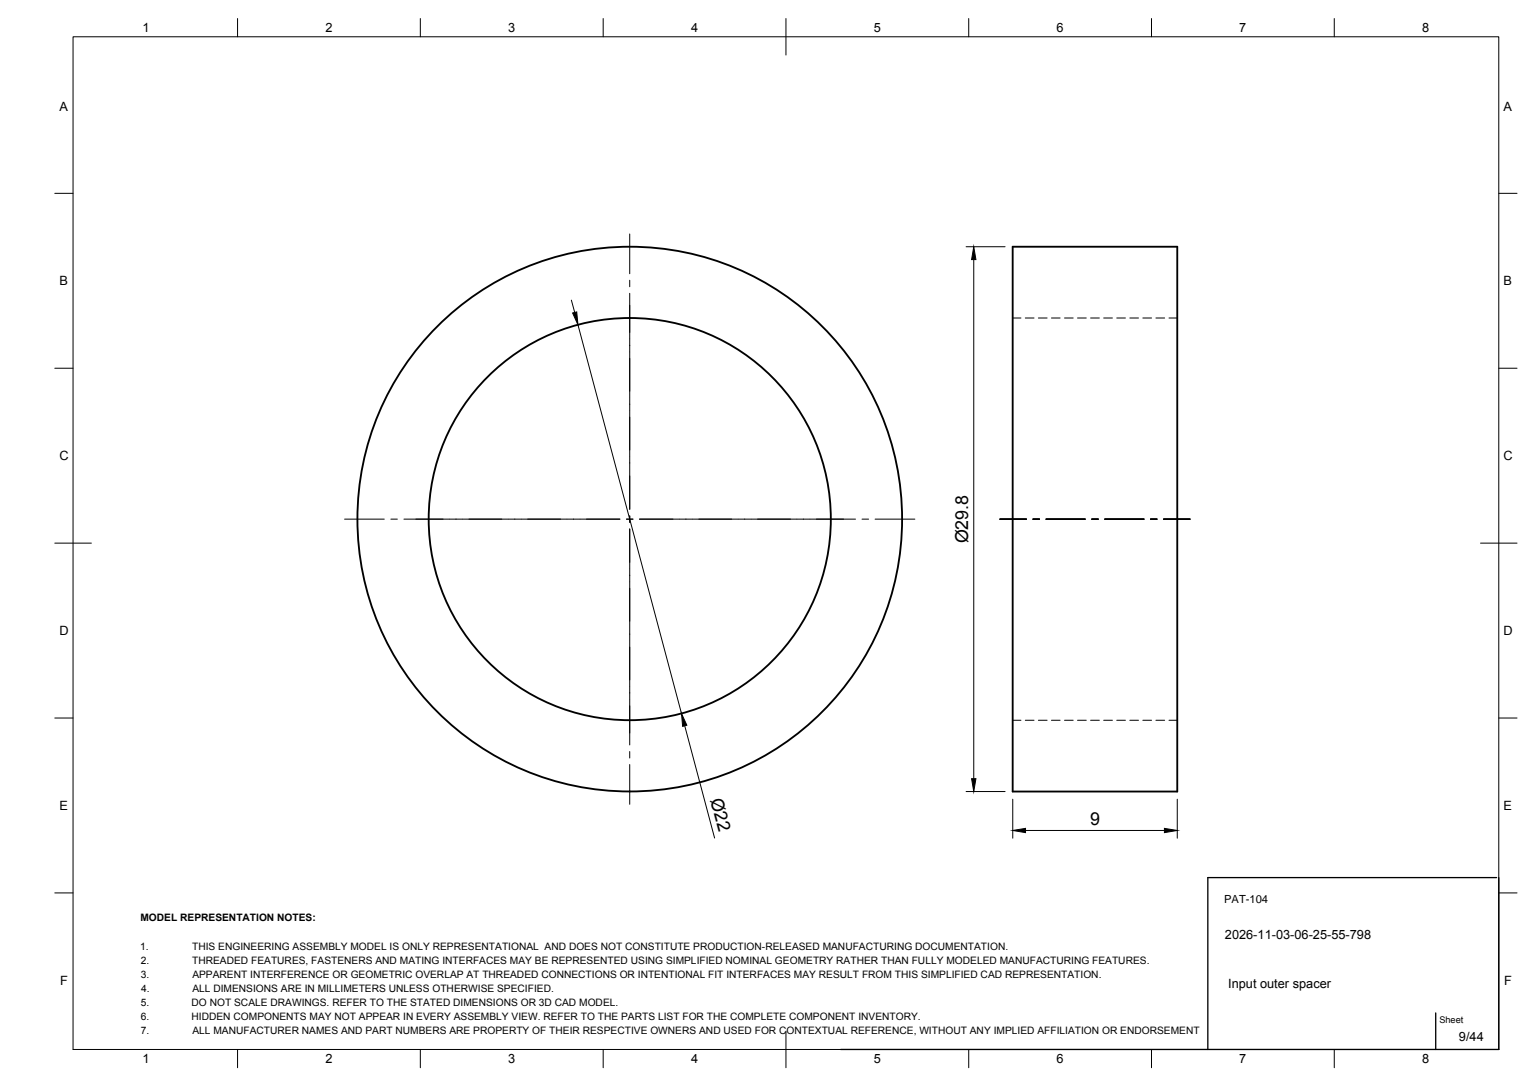
ISO-10303-21;
HEADER;
/* Generated by software containing ST-Developer
 * from STEP Tools, Inc. (www.steptools.com) 
 */

FILE_DESCRIPTION(
/* description */ ('Timing belt drive module 2 mm Pitch Timing 20T-40T'),

/* implementation_level */ '2;1');

FILE_NAME(
/* name */ 'Input outer spacer.step',
/* time_stamp */ '2026-10-28T03:25:12-07:00',
/* author */ (''),
/* organization */ (''),
/* preprocessor_version */ 'ST-DEVELOPER v20.2',
/* originating_system */ 'Autodesk Translation Framework v15.17.0.0',
/* authorisation */ '');

FILE_SCHEMA (('AUTOMOTIVE_DESIGN { 1 0 10303 214 3 1 1 }'));
ENDSEC;

DATA;
#10=MECHANICAL_DESIGN_GEOMETRIC_PRESENTATION_REPRESENTATION('',(#528),#17830);
#442=SHAPE_REPRESENTATION_RELATIONSHIP('SRR','None',#18012,#485);
#485=ADVANCED_BREP_SHAPE_REPRESENTATION('',(#586),#17787);
#528=STYLED_ITEM('',(#18310),#586);
#586=MANIFOLD_SOLID_BREP('Body1',#8985);
#665=FACE_BOUND('',#1575,.T.);
#666=FACE_BOUND('',#1577,.T.);
#813=PLANE('',#9636);
#814=PLANE('',#9637);
#1023=FACE_OUTER_BOUND('',#1572,.T.);
#1024=FACE_OUTER_BOUND('',#1573,.T.);
#1025=FACE_OUTER_BOUND('',#1574,.T.);
#1026=FACE_OUTER_BOUND('',#1576,.T.);
#1572=EDGE_LOOP('',(#6079,#6080,#6081,#6082));
#1573=EDGE_LOOP('',(#6083,#6084,#6085,#6086));
#1574=EDGE_LOOP('',(#6087));
#1575=EDGE_LOOP('',(#6088));
#1576=EDGE_LOOP('',(#6089));
#1577=EDGE_LOOP('',(#6090));
#2186=CIRCLE('',#9631,1.1);
#2187=CIRCLE('',#9632,1.1);
#2188=CIRCLE('',#9634,1.49);
#2189=CIRCLE('',#9635,1.49);
#2897=LINE('',#14200,#3375);
#2898=LINE('',#14206,#3376);
#3375=VECTOR('',#11148,1.1);
#3376=VECTOR('',#11155,1.49);
#3848=VERTEX_POINT('',#14197);
#3849=VERTEX_POINT('',#14199);
#3850=VERTEX_POINT('',#14203);
#3851=VERTEX_POINT('',#14205);
#4722=EDGE_CURVE('',#3848,#3848,#2186,.T.);
#4723=EDGE_CURVE('',#3848,#3849,#2897,.T.);
#4724=EDGE_CURVE('',#3849,#3849,#2187,.T.);
#4725=EDGE_CURVE('',#3850,#3850,#2188,.T.);
#4726=EDGE_CURVE('',#3850,#3851,#2898,.T.);
#4727=EDGE_CURVE('',#3851,#3851,#2189,.T.);
#6079=ORIENTED_EDGE('',*,*,#4722,.F.);
#6080=ORIENTED_EDGE('',*,*,#4723,.T.);
#6081=ORIENTED_EDGE('',*,*,#4724,.T.);
#6082=ORIENTED_EDGE('',*,*,#4723,.F.);
#6083=ORIENTED_EDGE('',*,*,#4725,.F.);
#6084=ORIENTED_EDGE('',*,*,#4726,.T.);
#6085=ORIENTED_EDGE('',*,*,#4727,.T.);
#6086=ORIENTED_EDGE('',*,*,#4726,.F.);
#6087=ORIENTED_EDGE('',*,*,#4725,.T.);
#6088=ORIENTED_EDGE('',*,*,#4722,.T.);
#6089=ORIENTED_EDGE('',*,*,#4727,.F.);
#6090=ORIENTED_EDGE('',*,*,#4724,.F.);
#8202=CYLINDRICAL_SURFACE('',#9630,1.1);
#8203=CYLINDRICAL_SURFACE('',#9633,1.49);
#8521=ADVANCED_FACE('',(#1023),#8202,.F.);
#8522=ADVANCED_FACE('',(#1024),#8203,.T.);
#8523=ADVANCED_FACE('',(#1025,#665),#813,.T.);
#8524=ADVANCED_FACE('',(#1026,#666),#814,.F.);
#8985=CLOSED_SHELL('',(#8521,#8522,#8523,#8524));
#9629=AXIS2_PLACEMENT_3D('',#14195,#11142,#11143);
#9630=AXIS2_PLACEMENT_3D('',#14196,#11144,#11145);
#9631=AXIS2_PLACEMENT_3D('',#14198,#11146,#11147);
#9632=AXIS2_PLACEMENT_3D('',#14201,#11149,#11150);
#9633=AXIS2_PLACEMENT_3D('',#14202,#11151,#11152);
#9634=AXIS2_PLACEMENT_3D('',#14204,#11153,#11154);
#9635=AXIS2_PLACEMENT_3D('',#14207,#11156,#11157);
#9636=AXIS2_PLACEMENT_3D('',#14208,#11158,#11159);
#9637=AXIS2_PLACEMENT_3D('',#14209,#11160,#11161);
#11142=DIRECTION('axis',(0.,0.,1.));
#11143=DIRECTION('refdir',(1.,0.,0.));
#11144=DIRECTION('center_axis',(0.,1.,0.));
#11145=DIRECTION('ref_axis',(1.,0.,0.));
#11146=DIRECTION('center_axis',(0.,-1.,0.));
#11147=DIRECTION('ref_axis',(1.,0.,0.));
#11148=DIRECTION('',(0.,-1.,0.));
#11149=DIRECTION('center_axis',(0.,-1.,0.));
#11150=DIRECTION('ref_axis',(1.,0.,0.));
#11151=DIRECTION('center_axis',(0.,1.,0.));
#11152=DIRECTION('ref_axis',(1.,0.,0.));
#11153=DIRECTION('center_axis',(0.,1.,0.));
#11154=DIRECTION('ref_axis',(1.,0.,0.));
#11155=DIRECTION('',(0.,-1.,0.));
#11156=DIRECTION('center_axis',(0.,1.,0.));
#11157=DIRECTION('ref_axis',(1.,0.,0.));
#11158=DIRECTION('center_axis',(0.,1.,0.));
#11159=DIRECTION('ref_axis',(1.,0.,0.));
#11160=DIRECTION('center_axis',(0.,1.,0.));
#11161=DIRECTION('ref_axis',(1.,0.,0.));
#14195=CARTESIAN_POINT('',(0.,0.,0.));
#14196=CARTESIAN_POINT('Origin',(0.,-0.45,7.));
#14197=CARTESIAN_POINT('',(-1.1,0.45,7.));
#14198=CARTESIAN_POINT('Origin',(0.,0.45,7.));
#14199=CARTESIAN_POINT('',(-1.1,-0.45,7.));
#14200=CARTESIAN_POINT('',(-1.1,-0.45,7.));
#14201=CARTESIAN_POINT('Origin',(0.,-0.45,7.));
#14202=CARTESIAN_POINT('Origin',(0.,-0.45,7.));
#14203=CARTESIAN_POINT('',(-1.49,0.45,7.));
#14204=CARTESIAN_POINT('Origin',(0.,0.45,7.));
#14205=CARTESIAN_POINT('',(-1.49,-0.45,7.));
#14206=CARTESIAN_POINT('',(-1.49,-0.45,7.));
#14207=CARTESIAN_POINT('Origin',(0.,-0.45,7.));
#14208=CARTESIAN_POINT('Origin',(0.,0.45,7.));
#14209=CARTESIAN_POINT('Origin',(0.,-0.45,7.));
#17737=UNCERTAINTY_MEASURE_WITH_UNIT(LENGTH_MEASURE(0.001),#17831,
'DISTANCE_ACCURACY_VALUE',
'Maximum model space distance between geometric entities at asserted c
onnectivities');
#17780=UNCERTAINTY_MEASURE_WITH_UNIT(LENGTH_MEASURE(0.001),#17831,
'DISTANCE_ACCURACY_VALUE',
'Maximum model space distance between geometric entities at asserted c
onnectivities');
#17787=(
GEOMETRIC_REPRESENTATION_CONTEXT(3)
GLOBAL_UNCERTAINTY_ASSIGNED_CONTEXT((#17737))
GLOBAL_UNIT_ASSIGNED_CONTEXT((#17831,#17833,#17834))
REPRESENTATION_CONTEXT('','3D')
);
#17830=(
GEOMETRIC_REPRESENTATION_CONTEXT(3)
GLOBAL_UNCERTAINTY_ASSIGNED_CONTEXT((#17780))
GLOBAL_UNIT_ASSIGNED_CONTEXT((#17831,#17833,#17834))
REPRESENTATION_CONTEXT('','3D')
);
#17831=(
LENGTH_UNIT()
NAMED_UNIT(*)
SI_UNIT(.CENTI.,.METRE.)
);
#17833=(
NAMED_UNIT(*)
PLANE_ANGLE_UNIT()
SI_UNIT($,.RADIAN.)
);
#17834=(
NAMED_UNIT(*)
SI_UNIT($,.STERADIAN.)
SOLID_ANGLE_UNIT()
);
#17841=SHAPE_DEFINITION_REPRESENTATION(#17890,#18012);
#17890=PRODUCT_DEFINITION_SHAPE('',$,#18062);
#18012=SHAPE_REPRESENTATION('',(#9629),#17787);
#18055=PRODUCT_DEFINITION_CONTEXT('part definition',#18204,'design');
#18062=PRODUCT_DEFINITION('Input outer spacer','Input outer spacer',#18111,
#18055);
#18111=PRODUCT_DEFINITION_FORMATION('',$,#18212);
#18204=APPLICATION_CONTEXT(
'Core Data for Automotive Mechanical Design Process');
#18205=PRODUCT_CONTEXT('part definition',#18204,'mechanical');
#18212=PRODUCT('Input outer spacer','Input outer spacer',
'Input outer spacer',(#18205));
#18304=COLOUR_RGB('Sky Blue',0.24,0.69,0.87);
#18305=FILL_AREA_STYLE_COLOUR('',#18304);
#18306=FILL_AREA_STYLE('',(#18305));
#18307=SURFACE_STYLE_FILL_AREA(#18306);
#18308=SURFACE_SIDE_STYLE('',(#18307));
#18309=SURFACE_STYLE_USAGE(.BOTH.,#18308);
#18310=PRESENTATION_STYLE_ASSIGNMENT((#18309));
ENDSEC;
END-ISO-10303-21;
